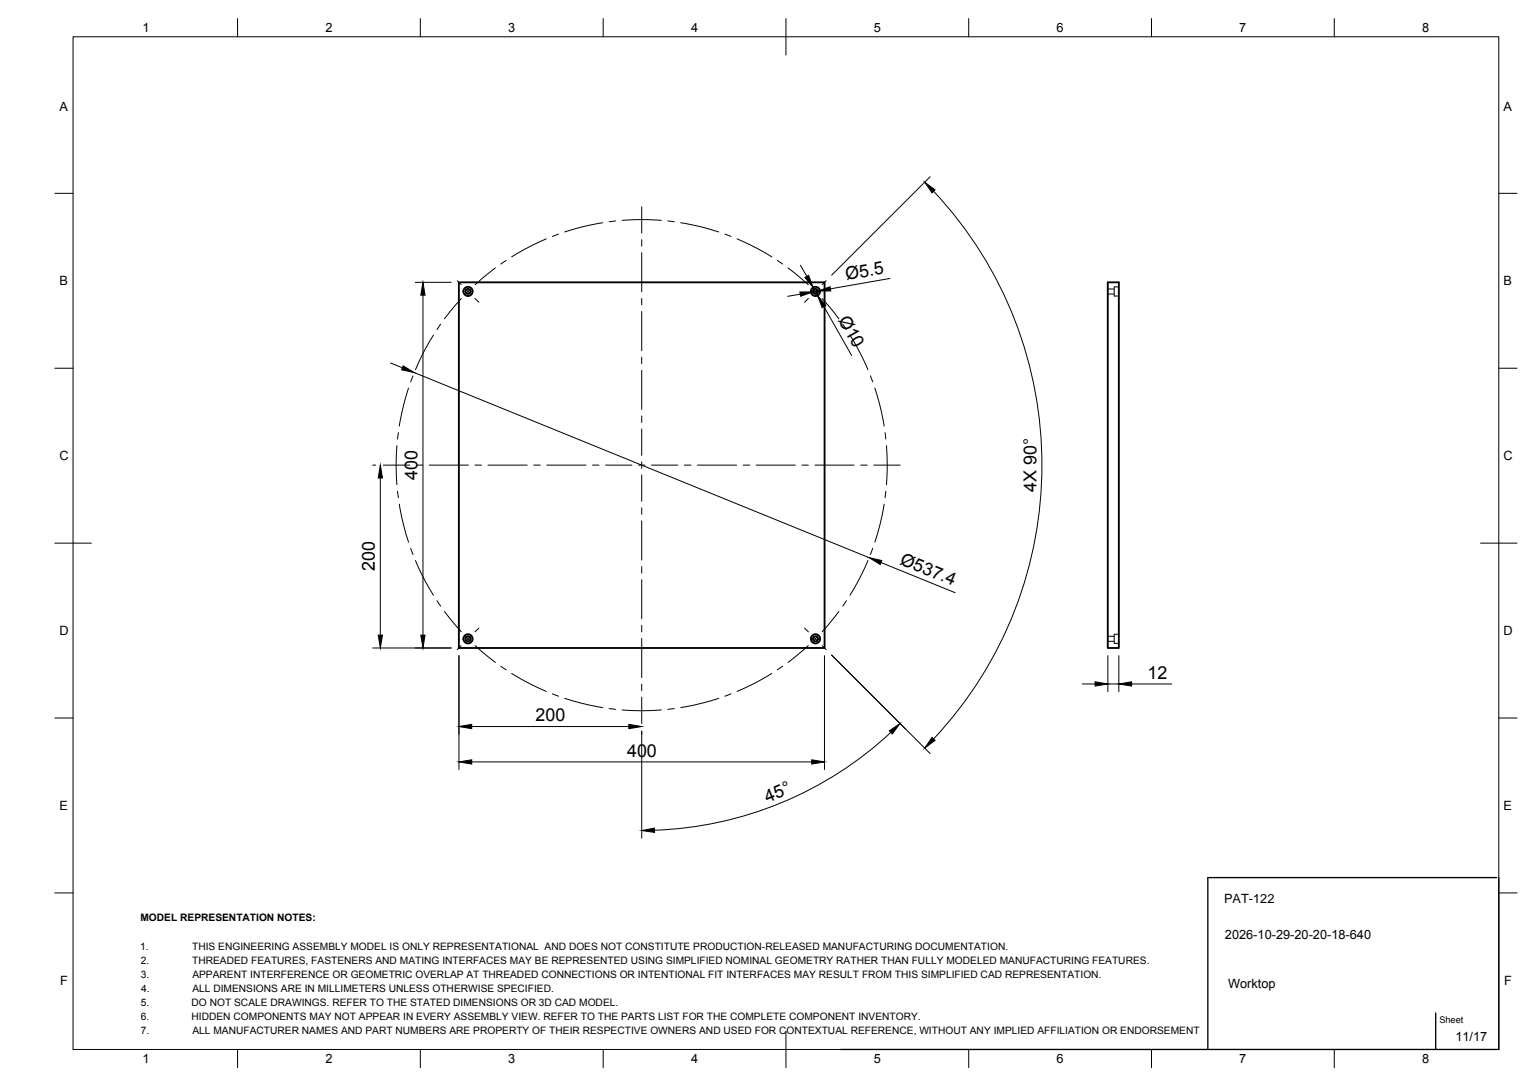
ISO-10303-21;
HEADER;
/* Generated by software containing ST-Developer
 * from STEP Tools, Inc. (www.steptools.com) 
 */

FILE_DESCRIPTION(
/* description */ ('PAT-122'),
/* implementation_level */ '2;1');

FILE_NAME(
/* name */ 'Worktop.step',
/* time_stamp */ '2026-10-29T20:20:12-07:00',
/* author */ (''),
/* organization */ (''),
/* preprocessor_version */ 'ST-DEVELOPER v20.2',
/* originating_system */ 'Autodesk Translation Framework v15.17.0.0',
/* authorisation */ '');

FILE_SCHEMA (('AUTOMOTIVE_DESIGN { 1 0 10303 214 3 1 1 }'));
ENDSEC;

DATA;
#10=MECHANICAL_DESIGN_GEOMETRIC_PRESENTATION_REPRESENTATION('',(#499),#10019);
#455=SHAPE_REPRESENTATION_RELATIONSHIP('SRR','None',#10176,#477);
#477=ADVANCED_BREP_SHAPE_REPRESENTATION('',(#521),#10005);
#499=STYLED_ITEM('',(#10341),#521);
#521=MANIFOLD_SOLID_BREP('Body1',#5621);
#547=FACE_BOUND('',#1167,.T.);
#548=FACE_BOUND('',#1170,.T.);
#549=FACE_BOUND('',#1173,.T.);
#550=FACE_BOUND('',#1176,.T.);
#551=FACE_BOUND('',#1186,.T.);
#552=FACE_BOUND('',#1187,.T.);
#553=FACE_BOUND('',#1188,.T.);
#554=FACE_BOUND('',#1189,.T.);
#555=FACE_BOUND('',#1191,.T.);
#556=FACE_BOUND('',#1192,.T.);
#557=FACE_BOUND('',#1193,.T.);
#558=FACE_BOUND('',#1194,.T.);
#625=PLANE('',#5959);
#626=PLANE('',#5964);
#627=PLANE('',#5969);
#628=PLANE('',#5974);
#629=PLANE('',#5984);
#630=PLANE('',#5985);
#631=PLANE('',#5986);
#632=PLANE('',#5987);
#633=PLANE('',#5988);
#634=PLANE('',#5989);
#857=FACE_OUTER_BOUND('',#1165,.T.);
#858=FACE_OUTER_BOUND('',#1166,.T.);
#859=FACE_OUTER_BOUND('',#1168,.T.);
#860=FACE_OUTER_BOUND('',#1169,.T.);
#861=FACE_OUTER_BOUND('',#1171,.T.);
#862=FACE_OUTER_BOUND('',#1172,.T.);
#863=FACE_OUTER_BOUND('',#1174,.T.);
#864=FACE_OUTER_BOUND('',#1175,.T.);
#865=FACE_OUTER_BOUND('',#1177,.T.);
#866=FACE_OUTER_BOUND('',#1178,.T.);
#867=FACE_OUTER_BOUND('',#1179,.T.);
#868=FACE_OUTER_BOUND('',#1180,.T.);
#869=FACE_OUTER_BOUND('',#1181,.T.);
#870=FACE_OUTER_BOUND('',#1182,.T.);
#871=FACE_OUTER_BOUND('',#1183,.T.);
#872=FACE_OUTER_BOUND('',#1184,.T.);
#873=FACE_OUTER_BOUND('',#1185,.T.);
#874=FACE_OUTER_BOUND('',#1190,.T.);
#1165=EDGE_LOOP('',(#3961,#3962,#3963,#3964));
#1166=EDGE_LOOP('',(#3965));
#1167=EDGE_LOOP('',(#3966));
#1168=EDGE_LOOP('',(#3967,#3968,#3969,#3970));
#1169=EDGE_LOOP('',(#3971));
#1170=EDGE_LOOP('',(#3972));
#1171=EDGE_LOOP('',(#3973,#3974,#3975,#3976));
#1172=EDGE_LOOP('',(#3977));
#1173=EDGE_LOOP('',(#3978));
#1174=EDGE_LOOP('',(#3979,#3980,#3981,#3982));
#1175=EDGE_LOOP('',(#3983));
#1176=EDGE_LOOP('',(#3984));
#1177=EDGE_LOOP('',(#3985,#3986,#3987,#3988));
#1178=EDGE_LOOP('',(#3989,#3990,#3991,#3992));
#1179=EDGE_LOOP('',(#3993,#3994,#3995,#3996));
#1180=EDGE_LOOP('',(#3997,#3998,#3999,#4000));
#1181=EDGE_LOOP('',(#4001,#4002,#4003,#4004));
#1182=EDGE_LOOP('',(#4005,#4006,#4007,#4008));
#1183=EDGE_LOOP('',(#4009,#4010,#4011,#4012));
#1184=EDGE_LOOP('',(#4013,#4014,#4015,#4016));
#1185=EDGE_LOOP('',(#4017,#4018,#4019,#4020));
#1186=EDGE_LOOP('',(#4021));
#1187=EDGE_LOOP('',(#4022));
#1188=EDGE_LOOP('',(#4023));
#1189=EDGE_LOOP('',(#4024));
#1190=EDGE_LOOP('',(#4025,#4026,#4027,#4028));
#1191=EDGE_LOOP('',(#4029));
#1192=EDGE_LOOP('',(#4030));
#1193=EDGE_LOOP('',(#4031));
#1194=EDGE_LOOP('',(#4032));
#1503=LINE('',#8184,#2047);
#1504=LINE('',#8193,#2048);
#1505=LINE('',#8202,#2049);
#1506=LINE('',#8211,#2050);
#1507=LINE('',#8219,#2051);
#1508=LINE('',#8223,#2052);
#1509=LINE('',#8227,#2053);
#1510=LINE('',#8231,#2054);
#1511=LINE('',#8235,#2055);
#1512=LINE('',#8237,#2056);
#1513=LINE('',#8239,#2057);
#1514=LINE('',#8240,#2058);
#1515=LINE('',#8243,#2059);
#1516=LINE('',#8245,#2060);
#1517=LINE('',#8246,#2061);
#1518=LINE('',#8249,#2062);
#1519=LINE('',#8251,#2063);
#1520=LINE('',#8252,#2064);
#1521=LINE('',#8254,#2065);
#1522=LINE('',#8255,#2066);
#2047=VECTOR('',#6594,0.5);
#2048=VECTOR('',#6605,0.5);
#2049=VECTOR('',#6616,0.5);
#2050=VECTOR('',#6627,0.5);
#2051=VECTOR('',#6638,0.274999999999999);
#2052=VECTOR('',#6643,0.274999999999999);
#2053=VECTOR('',#6648,0.274999999999999);
#2054=VECTOR('',#6653,0.274999999999999);
#2055=VECTOR('',#6656,1.);
#2056=VECTOR('',#6657,1.);
#2057=VECTOR('',#6658,1.);
#2058=VECTOR('',#6659,1.);
#2059=VECTOR('',#6662,1.);
#2060=VECTOR('',#6663,1.);
#2061=VECTOR('',#6664,1.);
#2062=VECTOR('',#6667,1.);
#2063=VECTOR('',#6668,1.);
#2064=VECTOR('',#6669,1.);
#2065=VECTOR('',#6672,1.);
#2066=VECTOR('',#6673,1.);
#2607=CIRCLE('',#5957,0.5);
#2608=CIRCLE('',#5958,0.5);
#2609=CIRCLE('',#5960,0.274999999999999);
#2610=CIRCLE('',#5962,0.5);
#2611=CIRCLE('',#5963,0.5);
#2612=CIRCLE('',#5965,0.274999999999999);
#2613=CIRCLE('',#5967,0.5);
#2614=CIRCLE('',#5968,0.5);
#2615=CIRCLE('',#5970,0.274999999999999);
#2616=CIRCLE('',#5972,0.5);
#2617=CIRCLE('',#5973,0.5);
#2618=CIRCLE('',#5975,0.274999999999999);
#2619=CIRCLE('',#5977,0.274999999999999);
#2620=CIRCLE('',#5979,0.274999999999999);
#2621=CIRCLE('',#5981,0.274999999999999);
#2622=CIRCLE('',#5983,0.274999999999999);
#2737=VERTEX_POINT('',#8181);
#2738=VERTEX_POINT('',#8183);
#2739=VERTEX_POINT('',#8187);
#2740=VERTEX_POINT('',#8190);
#2741=VERTEX_POINT('',#8192);
#2742=VERTEX_POINT('',#8196);
#2743=VERTEX_POINT('',#8199);
#2744=VERTEX_POINT('',#8201);
#2745=VERTEX_POINT('',#8205);
#2746=VERTEX_POINT('',#8208);
#2747=VERTEX_POINT('',#8210);
#2748=VERTEX_POINT('',#8214);
#2749=VERTEX_POINT('',#8217);
#2750=VERTEX_POINT('',#8221);
#2751=VERTEX_POINT('',#8225);
#2752=VERTEX_POINT('',#8229);
#2753=VERTEX_POINT('',#8233);
#2754=VERTEX_POINT('',#8234);
#2755=VERTEX_POINT('',#8236);
#2756=VERTEX_POINT('',#8238);
#2757=VERTEX_POINT('',#8242);
#2758=VERTEX_POINT('',#8244);
#2759=VERTEX_POINT('',#8248);
#2760=VERTEX_POINT('',#8250);
#3215=EDGE_CURVE('',#2737,#2737,#2607,.T.);
#3216=EDGE_CURVE('',#2737,#2738,#1503,.T.);
#3217=EDGE_CURVE('',#2738,#2738,#2608,.T.);
#3218=EDGE_CURVE('',#2739,#2739,#2609,.T.);
#3219=EDGE_CURVE('',#2740,#2740,#2610,.T.);
#3220=EDGE_CURVE('',#2740,#2741,#1504,.T.);
#3221=EDGE_CURVE('',#2741,#2741,#2611,.T.);
#3222=EDGE_CURVE('',#2742,#2742,#2612,.T.);
#3223=EDGE_CURVE('',#2743,#2743,#2613,.T.);
#3224=EDGE_CURVE('',#2743,#2744,#1505,.T.);
#3225=EDGE_CURVE('',#2744,#2744,#2614,.T.);
#3226=EDGE_CURVE('',#2745,#2745,#2615,.T.);
#3227=EDGE_CURVE('',#2746,#2746,#2616,.T.);
#3228=EDGE_CURVE('',#2746,#2747,#1506,.T.);
#3229=EDGE_CURVE('',#2747,#2747,#2617,.T.);
#3230=EDGE_CURVE('',#2748,#2748,#2618,.T.);
#3231=EDGE_CURVE('',#2749,#2749,#2619,.T.);
#3232=EDGE_CURVE('',#2749,#2739,#1507,.T.);
#3233=EDGE_CURVE('',#2750,#2750,#2620,.T.);
#3234=EDGE_CURVE('',#2750,#2742,#1508,.T.);
#3235=EDGE_CURVE('',#2751,#2751,#2621,.T.);
#3236=EDGE_CURVE('',#2751,#2745,#1509,.T.);
#3237=EDGE_CURVE('',#2752,#2752,#2622,.T.);
#3238=EDGE_CURVE('',#2752,#2748,#1510,.T.);
#3239=EDGE_CURVE('',#2753,#2754,#1511,.T.);
#3240=EDGE_CURVE('',#2754,#2755,#1512,.T.);
#3241=EDGE_CURVE('',#2756,#2755,#1513,.T.);
#3242=EDGE_CURVE('',#2753,#2756,#1514,.T.);
#3243=EDGE_CURVE('',#2757,#2753,#1515,.T.);
#3244=EDGE_CURVE('',#2758,#2756,#1516,.T.);
#3245=EDGE_CURVE('',#2757,#2758,#1517,.T.);
#3246=EDGE_CURVE('',#2759,#2757,#1518,.T.);
#3247=EDGE_CURVE('',#2760,#2758,#1519,.T.);
#3248=EDGE_CURVE('',#2759,#2760,#1520,.T.);
#3249=EDGE_CURVE('',#2754,#2759,#1521,.T.);
#3250=EDGE_CURVE('',#2755,#2760,#1522,.T.);
#3961=ORIENTED_EDGE('',*,*,#3215,.F.);
#3962=ORIENTED_EDGE('',*,*,#3216,.T.);
#3963=ORIENTED_EDGE('',*,*,#3217,.F.);
#3964=ORIENTED_EDGE('',*,*,#3216,.F.);
#3965=ORIENTED_EDGE('',*,*,#3215,.T.);
#3966=ORIENTED_EDGE('',*,*,#3218,.F.);
#3967=ORIENTED_EDGE('',*,*,#3219,.F.);
#3968=ORIENTED_EDGE('',*,*,#3220,.T.);
#3969=ORIENTED_EDGE('',*,*,#3221,.F.);
#3970=ORIENTED_EDGE('',*,*,#3220,.F.);
#3971=ORIENTED_EDGE('',*,*,#3219,.T.);
#3972=ORIENTED_EDGE('',*,*,#3222,.F.);
#3973=ORIENTED_EDGE('',*,*,#3223,.F.);
#3974=ORIENTED_EDGE('',*,*,#3224,.T.);
#3975=ORIENTED_EDGE('',*,*,#3225,.F.);
#3976=ORIENTED_EDGE('',*,*,#3224,.F.);
#3977=ORIENTED_EDGE('',*,*,#3223,.T.);
#3978=ORIENTED_EDGE('',*,*,#3226,.F.);
#3979=ORIENTED_EDGE('',*,*,#3227,.F.);
#3980=ORIENTED_EDGE('',*,*,#3228,.T.);
#3981=ORIENTED_EDGE('',*,*,#3229,.F.);
#3982=ORIENTED_EDGE('',*,*,#3228,.F.);
#3983=ORIENTED_EDGE('',*,*,#3227,.T.);
#3984=ORIENTED_EDGE('',*,*,#3230,.F.);
#3985=ORIENTED_EDGE('',*,*,#3231,.F.);
#3986=ORIENTED_EDGE('',*,*,#3232,.T.);
#3987=ORIENTED_EDGE('',*,*,#3218,.T.);
#3988=ORIENTED_EDGE('',*,*,#3232,.F.);
#3989=ORIENTED_EDGE('',*,*,#3233,.F.);
#3990=ORIENTED_EDGE('',*,*,#3234,.T.);
#3991=ORIENTED_EDGE('',*,*,#3222,.T.);
#3992=ORIENTED_EDGE('',*,*,#3234,.F.);
#3993=ORIENTED_EDGE('',*,*,#3235,.F.);
#3994=ORIENTED_EDGE('',*,*,#3236,.T.);
#3995=ORIENTED_EDGE('',*,*,#3226,.T.);
#3996=ORIENTED_EDGE('',*,*,#3236,.F.);
#3997=ORIENTED_EDGE('',*,*,#3237,.F.);
#3998=ORIENTED_EDGE('',*,*,#3238,.T.);
#3999=ORIENTED_EDGE('',*,*,#3230,.T.);
#4000=ORIENTED_EDGE('',*,*,#3238,.F.);
#4001=ORIENTED_EDGE('',*,*,#3239,.T.);
#4002=ORIENTED_EDGE('',*,*,#3240,.T.);
#4003=ORIENTED_EDGE('',*,*,#3241,.F.);
#4004=ORIENTED_EDGE('',*,*,#3242,.F.);
#4005=ORIENTED_EDGE('',*,*,#3243,.T.);
#4006=ORIENTED_EDGE('',*,*,#3242,.T.);
#4007=ORIENTED_EDGE('',*,*,#3244,.F.);
#4008=ORIENTED_EDGE('',*,*,#3245,.F.);
#4009=ORIENTED_EDGE('',*,*,#3246,.T.);
#4010=ORIENTED_EDGE('',*,*,#3245,.T.);
#4011=ORIENTED_EDGE('',*,*,#3247,.F.);
#4012=ORIENTED_EDGE('',*,*,#3248,.F.);
#4013=ORIENTED_EDGE('',*,*,#3249,.T.);
#4014=ORIENTED_EDGE('',*,*,#3248,.T.);
#4015=ORIENTED_EDGE('',*,*,#3250,.F.);
#4016=ORIENTED_EDGE('',*,*,#3240,.F.);
#4017=ORIENTED_EDGE('',*,*,#3250,.T.);
#4018=ORIENTED_EDGE('',*,*,#3247,.T.);
#4019=ORIENTED_EDGE('',*,*,#3244,.T.);
#4020=ORIENTED_EDGE('',*,*,#3241,.T.);
#4021=ORIENTED_EDGE('',*,*,#3229,.T.);
#4022=ORIENTED_EDGE('',*,*,#3225,.T.);
#4023=ORIENTED_EDGE('',*,*,#3221,.T.);
#4024=ORIENTED_EDGE('',*,*,#3217,.T.);
#4025=ORIENTED_EDGE('',*,*,#3249,.F.);
#4026=ORIENTED_EDGE('',*,*,#3239,.F.);
#4027=ORIENTED_EDGE('',*,*,#3243,.F.);
#4028=ORIENTED_EDGE('',*,*,#3246,.F.);
#4029=ORIENTED_EDGE('',*,*,#3231,.T.);
#4030=ORIENTED_EDGE('',*,*,#3233,.T.);
#4031=ORIENTED_EDGE('',*,*,#3235,.T.);
#4032=ORIENTED_EDGE('',*,*,#3237,.T.);
#5277=CYLINDRICAL_SURFACE('',#5956,0.5);
#5278=CYLINDRICAL_SURFACE('',#5961,0.5);
#5279=CYLINDRICAL_SURFACE('',#5966,0.5);
#5280=CYLINDRICAL_SURFACE('',#5971,0.5);
#5281=CYLINDRICAL_SURFACE('',#5976,0.274999999999999);
#5282=CYLINDRICAL_SURFACE('',#5978,0.274999999999999);
#5283=CYLINDRICAL_SURFACE('',#5980,0.274999999999999);
#5284=CYLINDRICAL_SURFACE('',#5982,0.274999999999999);
#5353=ADVANCED_FACE('',(#857),#5277,.F.);
#5354=ADVANCED_FACE('',(#858,#547),#625,.T.);
#5355=ADVANCED_FACE('',(#859),#5278,.F.);
#5356=ADVANCED_FACE('',(#860,#548),#626,.T.);
#5357=ADVANCED_FACE('',(#861),#5279,.F.);
#5358=ADVANCED_FACE('',(#862,#549),#627,.T.);
#5359=ADVANCED_FACE('',(#863),#5280,.F.);
#5360=ADVANCED_FACE('',(#864,#550),#628,.T.);
#5361=ADVANCED_FACE('',(#865),#5281,.F.);
#5362=ADVANCED_FACE('',(#866),#5282,.F.);
#5363=ADVANCED_FACE('',(#867),#5283,.F.);
#5364=ADVANCED_FACE('',(#868),#5284,.F.);
#5365=ADVANCED_FACE('',(#869),#629,.T.);
#5366=ADVANCED_FACE('',(#870),#630,.T.);
#5367=ADVANCED_FACE('',(#871),#631,.T.);
#5368=ADVANCED_FACE('',(#872),#632,.T.);
#5369=ADVANCED_FACE('',(#873,#551,#552,#553,#554),#633,.T.);
#5370=ADVANCED_FACE('',(#874,#555,#556,#557,#558),#634,.F.);
#5621=CLOSED_SHELL('',(#5353,#5354,#5355,#5356,#5357,#5358,#5359,#5360,
#5361,#5362,#5363,#5364,#5365,#5366,#5367,#5368,#5369,#5370));
#5955=AXIS2_PLACEMENT_3D('',#8179,#6588,#6589);
#5956=AXIS2_PLACEMENT_3D('',#8180,#6590,#6591);
#5957=AXIS2_PLACEMENT_3D('',#8182,#6592,#6593);
#5958=AXIS2_PLACEMENT_3D('',#8185,#6595,#6596);
#5959=AXIS2_PLACEMENT_3D('',#8186,#6597,#6598);
#5960=AXIS2_PLACEMENT_3D('',#8188,#6599,#6600);
#5961=AXIS2_PLACEMENT_3D('',#8189,#6601,#6602);
#5962=AXIS2_PLACEMENT_3D('',#8191,#6603,#6604);
#5963=AXIS2_PLACEMENT_3D('',#8194,#6606,#6607);
#5964=AXIS2_PLACEMENT_3D('',#8195,#6608,#6609);
#5965=AXIS2_PLACEMENT_3D('',#8197,#6610,#6611);
#5966=AXIS2_PLACEMENT_3D('',#8198,#6612,#6613);
#5967=AXIS2_PLACEMENT_3D('',#8200,#6614,#6615);
#5968=AXIS2_PLACEMENT_3D('',#8203,#6617,#6618);
#5969=AXIS2_PLACEMENT_3D('',#8204,#6619,#6620);
#5970=AXIS2_PLACEMENT_3D('',#8206,#6621,#6622);
#5971=AXIS2_PLACEMENT_3D('',#8207,#6623,#6624);
#5972=AXIS2_PLACEMENT_3D('',#8209,#6625,#6626);
#5973=AXIS2_PLACEMENT_3D('',#8212,#6628,#6629);
#5974=AXIS2_PLACEMENT_3D('',#8213,#6630,#6631);
#5975=AXIS2_PLACEMENT_3D('',#8215,#6632,#6633);
#5976=AXIS2_PLACEMENT_3D('',#8216,#6634,#6635);
#5977=AXIS2_PLACEMENT_3D('',#8218,#6636,#6637);
#5978=AXIS2_PLACEMENT_3D('',#8220,#6639,#6640);
#5979=AXIS2_PLACEMENT_3D('',#8222,#6641,#6642);
#5980=AXIS2_PLACEMENT_3D('',#8224,#6644,#6645);
#5981=AXIS2_PLACEMENT_3D('',#8226,#6646,#6647);
#5982=AXIS2_PLACEMENT_3D('',#8228,#6649,#6650);
#5983=AXIS2_PLACEMENT_3D('',#8230,#6651,#6652);
#5984=AXIS2_PLACEMENT_3D('',#8232,#6654,#6655);
#5985=AXIS2_PLACEMENT_3D('',#8241,#6660,#6661);
#5986=AXIS2_PLACEMENT_3D('',#8247,#6665,#6666);
#5987=AXIS2_PLACEMENT_3D('',#8253,#6670,#6671);
#5988=AXIS2_PLACEMENT_3D('',#8256,#6674,#6675);
#5989=AXIS2_PLACEMENT_3D('',#8257,#6676,#6677);
#6588=DIRECTION('axis',(0.,0.,1.));
#6589=DIRECTION('refdir',(1.,0.,0.));
#6590=DIRECTION('center_axis',(0.,0.,1.));
#6591=DIRECTION('ref_axis',(1.,0.,0.));
#6592=DIRECTION('center_axis',(0.,0.,1.));
#6593=DIRECTION('ref_axis',(1.,0.,0.));
#6594=DIRECTION('',(0.,0.,1.));
#6595=DIRECTION('center_axis',(0.,0.,-1.));
#6596=DIRECTION('ref_axis',(1.,0.,0.));
#6597=DIRECTION('center_axis',(0.,0.,1.));
#6598=DIRECTION('ref_axis',(1.,0.,0.));
#6599=DIRECTION('center_axis',(0.,0.,1.));
#6600=DIRECTION('ref_axis',(1.,0.,0.));
#6601=DIRECTION('center_axis',(0.,0.,1.));
#6602=DIRECTION('ref_axis',(1.,0.,0.));
#6603=DIRECTION('center_axis',(0.,0.,1.));
#6604=DIRECTION('ref_axis',(1.,0.,0.));
#6605=DIRECTION('',(0.,0.,1.));
#6606=DIRECTION('center_axis',(0.,0.,-1.));
#6607=DIRECTION('ref_axis',(1.,0.,0.));
#6608=DIRECTION('center_axis',(0.,0.,1.));
#6609=DIRECTION('ref_axis',(1.,0.,0.));
#6610=DIRECTION('center_axis',(0.,0.,1.));
#6611=DIRECTION('ref_axis',(1.,0.,0.));
#6612=DIRECTION('center_axis',(0.,0.,1.));
#6613=DIRECTION('ref_axis',(1.,0.,0.));
#6614=DIRECTION('center_axis',(0.,0.,1.));
#6615=DIRECTION('ref_axis',(1.,0.,0.));
#6616=DIRECTION('',(0.,0.,1.));
#6617=DIRECTION('center_axis',(0.,0.,-1.));
#6618=DIRECTION('ref_axis',(1.,0.,0.));
#6619=DIRECTION('center_axis',(0.,0.,1.));
#6620=DIRECTION('ref_axis',(1.,0.,0.));
#6621=DIRECTION('center_axis',(0.,0.,1.));
#6622=DIRECTION('ref_axis',(1.,0.,0.));
#6623=DIRECTION('center_axis',(0.,0.,1.));
#6624=DIRECTION('ref_axis',(1.,0.,0.));
#6625=DIRECTION('center_axis',(0.,0.,1.));
#6626=DIRECTION('ref_axis',(1.,0.,0.));
#6627=DIRECTION('',(0.,0.,1.));
#6628=DIRECTION('center_axis',(0.,0.,-1.));
#6629=DIRECTION('ref_axis',(1.,0.,0.));
#6630=DIRECTION('center_axis',(0.,0.,1.));
#6631=DIRECTION('ref_axis',(1.,0.,0.));
#6632=DIRECTION('center_axis',(0.,0.,1.));
#6633=DIRECTION('ref_axis',(1.,0.,0.));
#6634=DIRECTION('center_axis',(0.,0.,1.));
#6635=DIRECTION('ref_axis',(1.,0.,0.));
#6636=DIRECTION('center_axis',(0.,0.,1.));
#6637=DIRECTION('ref_axis',(1.,0.,0.));
#6638=DIRECTION('',(0.,0.,1.));
#6639=DIRECTION('center_axis',(0.,0.,1.));
#6640=DIRECTION('ref_axis',(1.,0.,0.));
#6641=DIRECTION('center_axis',(0.,0.,1.));
#6642=DIRECTION('ref_axis',(1.,0.,0.));
#6643=DIRECTION('',(0.,0.,1.));
#6644=DIRECTION('center_axis',(0.,0.,1.));
#6645=DIRECTION('ref_axis',(1.,0.,0.));
#6646=DIRECTION('center_axis',(0.,0.,1.));
#6647=DIRECTION('ref_axis',(1.,0.,0.));
#6648=DIRECTION('',(0.,0.,1.));
#6649=DIRECTION('center_axis',(0.,0.,1.));
#6650=DIRECTION('ref_axis',(1.,0.,0.));
#6651=DIRECTION('center_axis',(0.,0.,1.));
#6652=DIRECTION('ref_axis',(1.,0.,0.));
#6653=DIRECTION('',(0.,0.,1.));
#6654=DIRECTION('center_axis',(0.,1.,0.));
#6655=DIRECTION('ref_axis',(-1.,0.,0.));
#6656=DIRECTION('',(-1.,0.,0.));
#6657=DIRECTION('',(0.,0.,1.));
#6658=DIRECTION('',(-1.,0.,0.));
#6659=DIRECTION('',(0.,0.,1.));
#6660=DIRECTION('center_axis',(1.,0.,0.));
#6661=DIRECTION('ref_axis',(0.,1.,0.));
#6662=DIRECTION('',(0.,1.,0.));
#6663=DIRECTION('',(0.,1.,0.));
#6664=DIRECTION('',(0.,0.,1.));
#6665=DIRECTION('center_axis',(0.,-1.,0.));
#6666=DIRECTION('ref_axis',(1.,0.,0.));
#6667=DIRECTION('',(1.,0.,0.));
#6668=DIRECTION('',(1.,0.,0.));
#6669=DIRECTION('',(0.,0.,1.));
#6670=DIRECTION('center_axis',(-1.,0.,0.));
#6671=DIRECTION('ref_axis',(0.,-1.,0.));
#6672=DIRECTION('',(0.,-1.,0.));
#6673=DIRECTION('',(0.,-1.,0.));
#6674=DIRECTION('center_axis',(0.,0.,1.));
#6675=DIRECTION('ref_axis',(1.,0.,0.));
#6676=DIRECTION('center_axis',(0.,0.,1.));
#6677=DIRECTION('ref_axis',(1.,0.,0.));
#8179=CARTESIAN_POINT('',(0.,0.,0.));
#8180=CARTESIAN_POINT('Origin',(19.,-19.,40.7));
#8181=CARTESIAN_POINT('',(18.5,-19.,40.7));
#8182=CARTESIAN_POINT('Origin',(19.,-19.,40.7));
#8183=CARTESIAN_POINT('',(18.5,-19.,41.2));
#8184=CARTESIAN_POINT('',(18.5,-19.,40.7));
#8185=CARTESIAN_POINT('Origin',(19.,-19.,41.2));
#8186=CARTESIAN_POINT('Origin',(19.,-19.,40.7));
#8187=CARTESIAN_POINT('',(18.725,-19.,40.7));
#8188=CARTESIAN_POINT('Origin',(19.,-19.,40.7));
#8189=CARTESIAN_POINT('Origin',(-19.,19.,40.7));
#8190=CARTESIAN_POINT('',(-19.5,19.,40.7));
#8191=CARTESIAN_POINT('Origin',(-19.,19.,40.7));
#8192=CARTESIAN_POINT('',(-19.5,19.,41.2));
#8193=CARTESIAN_POINT('',(-19.5,19.,40.7));
#8194=CARTESIAN_POINT('Origin',(-19.,19.,41.2));
#8195=CARTESIAN_POINT('Origin',(-19.,19.,40.7));
#8196=CARTESIAN_POINT('',(-19.275,19.,40.7));
#8197=CARTESIAN_POINT('Origin',(-19.,19.,40.7));
#8198=CARTESIAN_POINT('Origin',(-19.,-19.,40.7));
#8199=CARTESIAN_POINT('',(-19.5,-19.,40.7));
#8200=CARTESIAN_POINT('Origin',(-19.,-19.,40.7));
#8201=CARTESIAN_POINT('',(-19.5,-19.,41.2));
#8202=CARTESIAN_POINT('',(-19.5,-19.,40.7));
#8203=CARTESIAN_POINT('Origin',(-19.,-19.,41.2));
#8204=CARTESIAN_POINT('Origin',(-19.,-19.,40.7));
#8205=CARTESIAN_POINT('',(-19.275,-19.,40.7));
#8206=CARTESIAN_POINT('Origin',(-19.,-19.,40.7));
#8207=CARTESIAN_POINT('Origin',(19.,19.,40.7));
#8208=CARTESIAN_POINT('',(18.5,19.,40.7));
#8209=CARTESIAN_POINT('Origin',(19.,19.,40.7));
#8210=CARTESIAN_POINT('',(18.5,19.,41.2));
#8211=CARTESIAN_POINT('',(18.5,19.,40.7));
#8212=CARTESIAN_POINT('Origin',(19.,19.,41.2));
#8213=CARTESIAN_POINT('Origin',(19.,19.,40.7));
#8214=CARTESIAN_POINT('',(18.725,19.,40.7));
#8215=CARTESIAN_POINT('Origin',(19.,19.,40.7));
#8216=CARTESIAN_POINT('Origin',(19.,-19.,39.9));
#8217=CARTESIAN_POINT('',(18.725,-19.,40.));
#8218=CARTESIAN_POINT('Origin',(19.,-19.,40.));
#8219=CARTESIAN_POINT('',(18.725,-19.,39.9));
#8220=CARTESIAN_POINT('Origin',(-19.,19.,39.9));
#8221=CARTESIAN_POINT('',(-19.275,19.,40.));
#8222=CARTESIAN_POINT('Origin',(-19.,19.,40.));
#8223=CARTESIAN_POINT('',(-19.275,19.,39.9));
#8224=CARTESIAN_POINT('Origin',(-19.,-19.,39.9));
#8225=CARTESIAN_POINT('',(-19.275,-19.,40.));
#8226=CARTESIAN_POINT('Origin',(-19.,-19.,40.));
#8227=CARTESIAN_POINT('',(-19.275,-19.,39.9));
#8228=CARTESIAN_POINT('Origin',(19.,19.,39.9));
#8229=CARTESIAN_POINT('',(18.725,19.,40.));
#8230=CARTESIAN_POINT('Origin',(19.,19.,40.));
#8231=CARTESIAN_POINT('',(18.725,19.,39.9));
#8232=CARTESIAN_POINT('Origin',(20.,20.,40.));
#8233=CARTESIAN_POINT('',(20.,20.,40.));
#8234=CARTESIAN_POINT('',(-20.,20.,40.));
#8235=CARTESIAN_POINT('',(20.,20.,40.));
#8236=CARTESIAN_POINT('',(-20.,20.,41.2));
#8237=CARTESIAN_POINT('',(-20.,20.,40.));
#8238=CARTESIAN_POINT('',(20.,20.,41.2));
#8239=CARTESIAN_POINT('',(20.,20.,41.2));
#8240=CARTESIAN_POINT('',(20.,20.,40.));
#8241=CARTESIAN_POINT('Origin',(20.,-20.,40.));
#8242=CARTESIAN_POINT('',(20.,-20.,40.));
#8243=CARTESIAN_POINT('',(20.,-20.,40.));
#8244=CARTESIAN_POINT('',(20.,-20.,41.2));
#8245=CARTESIAN_POINT('',(20.,-20.,41.2));
#8246=CARTESIAN_POINT('',(20.,-20.,40.));
#8247=CARTESIAN_POINT('Origin',(-20.,-20.,40.));
#8248=CARTESIAN_POINT('',(-20.,-20.,40.));
#8249=CARTESIAN_POINT('',(-20.,-20.,40.));
#8250=CARTESIAN_POINT('',(-20.,-20.,41.2));
#8251=CARTESIAN_POINT('',(-20.,-20.,41.2));
#8252=CARTESIAN_POINT('',(-20.,-20.,40.));
#8253=CARTESIAN_POINT('Origin',(-20.,20.,40.));
#8254=CARTESIAN_POINT('',(-20.,20.,40.));
#8255=CARTESIAN_POINT('',(-20.,20.,41.2));
#8256=CARTESIAN_POINT('Origin',(0.,0.,41.2));
#8257=CARTESIAN_POINT('Origin',(0.,0.,40.));
#9981=UNCERTAINTY_MEASURE_WITH_UNIT(LENGTH_MEASURE(0.001),#10020,
'DISTANCE_ACCURACY_VALUE',
'Maximum model space distance between geometric entities at asserted c
onnectivities');
#9995=UNCERTAINTY_MEASURE_WITH_UNIT(LENGTH_MEASURE(0.001),#10020,
'DISTANCE_ACCURACY_VALUE',
'Maximum model space distance between geometric entities at asserted c
onnectivities');
#10005=(
GEOMETRIC_REPRESENTATION_CONTEXT(3)
GLOBAL_UNCERTAINTY_ASSIGNED_CONTEXT((#9981))
GLOBAL_UNIT_ASSIGNED_CONTEXT((#10020,#10022,#10023))
REPRESENTATION_CONTEXT('','3D')
);
#10019=(
GEOMETRIC_REPRESENTATION_CONTEXT(3)
GLOBAL_UNCERTAINTY_ASSIGNED_CONTEXT((#9995))
GLOBAL_UNIT_ASSIGNED_CONTEXT((#10020,#10022,#10023))
REPRESENTATION_CONTEXT('','3D')
);
#10020=(
LENGTH_UNIT()
NAMED_UNIT(*)
SI_UNIT(.CENTI.,.METRE.)
);
#10022=(
NAMED_UNIT(*)
PLANE_ANGLE_UNIT()
SI_UNIT($,.RADIAN.)
);
#10023=(
NAMED_UNIT(*)
SI_UNIT($,.STERADIAN.)
SOLID_ANGLE_UNIT()
);
#10033=SHAPE_DEFINITION_REPRESENTATION(#10056,#10176);
#10056=PRODUCT_DEFINITION_SHAPE('',$,#10200);
#10176=SHAPE_REPRESENTATION('',(#5955),#10005);
#10190=PRODUCT_DEFINITION_CONTEXT('part definition',#10261,'design');
#10200=PRODUCT_DEFINITION('Worktop','Worktop',#10223,#10190);
#10223=PRODUCT_DEFINITION_FORMATION('',$,#10272);
#10261=APPLICATION_CONTEXT(
'Core Data for Automotive Mechanical Design Process');
#10262=PRODUCT_CONTEXT('part definition',#10261,'mechanical');
#10272=PRODUCT('Worktop','Worktop','Worktop',(#10262));
#10335=COLOUR_RGB('Sky Blue',0.24,0.69,0.87);
#10336=FILL_AREA_STYLE_COLOUR('',#10335);
#10337=FILL_AREA_STYLE('',(#10336));
#10338=SURFACE_STYLE_FILL_AREA(#10337);
#10339=SURFACE_SIDE_STYLE('',(#10338));
#10340=SURFACE_STYLE_USAGE(.BOTH.,#10339);
#10341=PRESENTATION_STYLE_ASSIGNMENT((#10340));
ENDSEC;
END-ISO-10303-21;
